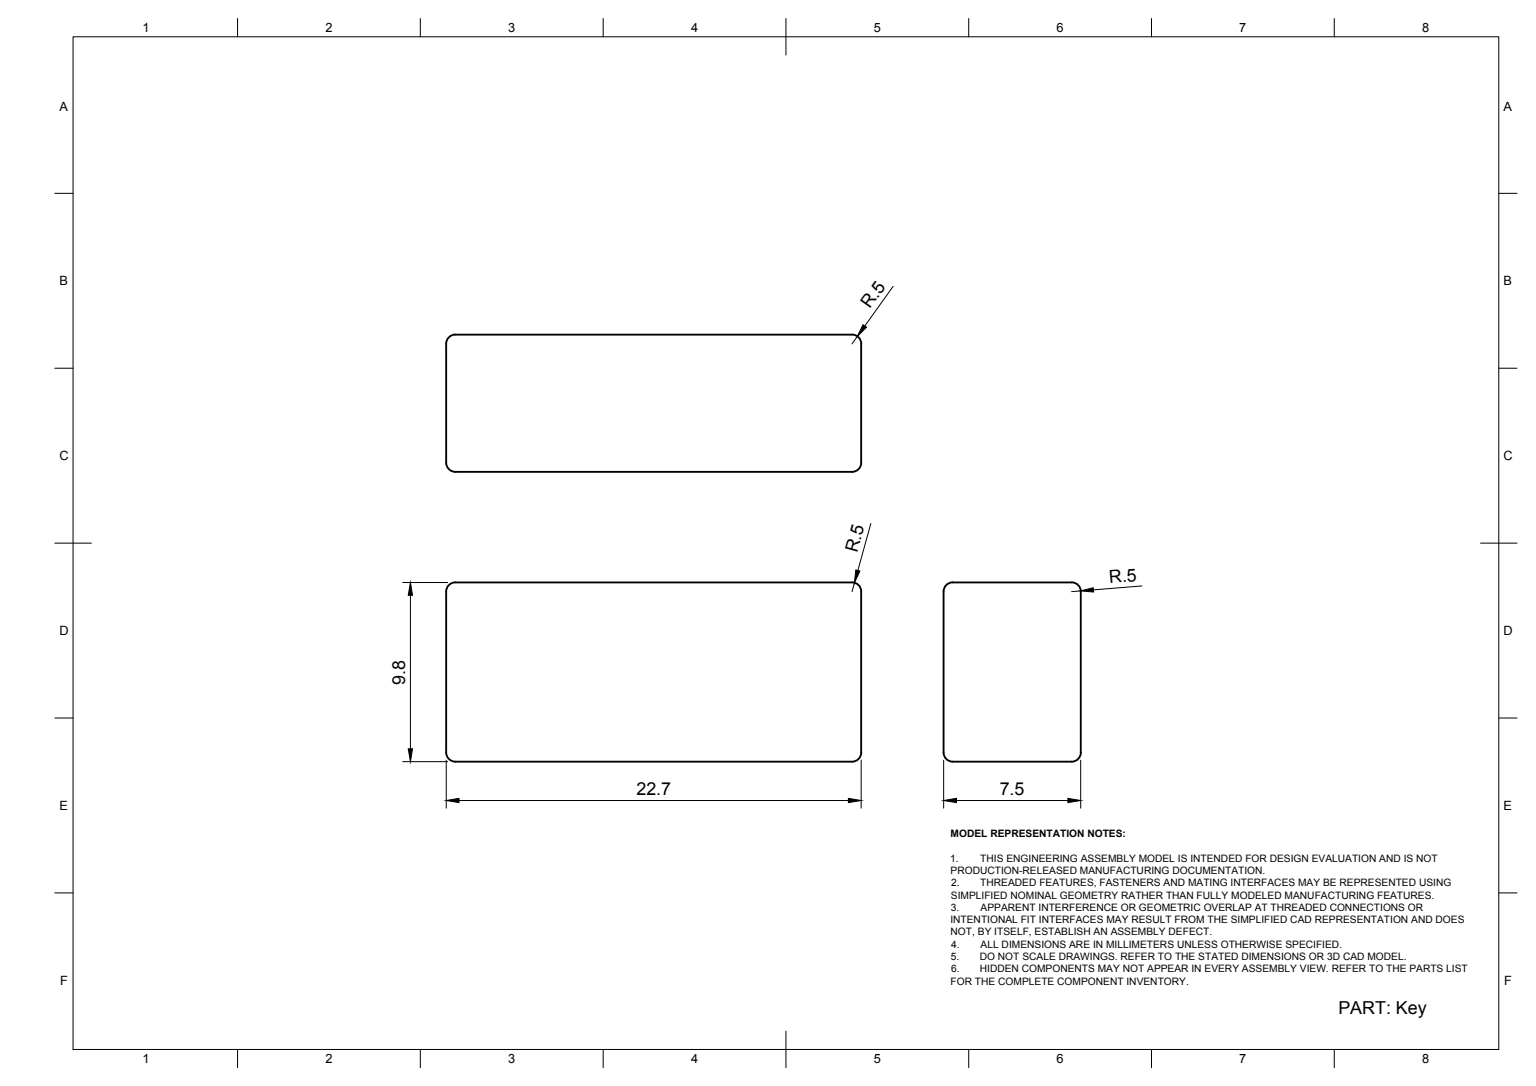
ISO-10303-21;
HEADER;
/* Generated by software containing ST-Developer
 * from STEP Tools, Inc. (www.steptools.com) 
 */

FILE_DESCRIPTION(
/* description */ ('STEP AP214'),
/* implementation_level */ '2;1');

FILE_NAME(
/* name */ 'Key.step',
/* time_stamp */ '2026-10-05T13:15:56-07:00',
/* author */ (''),
/* organization */ (''),
/* preprocessor_version */ 'ST-DEVELOPER v20.2',
/* originating_system */ 'Autodesk Translation Framework v15.15.0.0',
/* authorisation */ '');

FILE_SCHEMA (('AUTOMOTIVE_DESIGN { 1 0 10303 214 3 1 1 }'));
ENDSEC;

DATA;
#10=MECHANICAL_DESIGN_GEOMETRIC_PRESENTATION_REPRESENTATION('',(#1350),#37881);
#175=SPHERICAL_SURFACE('',#11699,0.5);
#176=SPHERICAL_SURFACE('',#11702,0.5);
#177=SPHERICAL_SURFACE('',#11719,0.5);
#178=SPHERICAL_SURFACE('',#11721,0.5);
#179=SPHERICAL_SURFACE('',#11723,0.5);
#180=SPHERICAL_SURFACE('',#11725,0.5);
#181=SPHERICAL_SURFACE('',#11735,0.5);
#182=SPHERICAL_SURFACE('',#11737,0.5);
#1326=SHAPE_REPRESENTATION_RELATIONSHIP('SRR','None',#37959,#1338);
#1338=ADVANCED_BREP_SHAPE_REPRESENTATION('',(#1362),#37874);
#1350=STYLED_ITEM('',(#38023),#1362);
#1362=MANIFOLD_SOLID_BREP('Body1',#10824);
#1525=PLANE('',#11690);
#1526=PLANE('',#11691);
#1527=PLANE('',#11692);
#1528=PLANE('',#11693);
#1529=PLANE('',#11694);
#1530=PLANE('',#11695);
#2091=FACE_OUTER_BOUND('',#2756,.T.);
#2092=FACE_OUTER_BOUND('',#2757,.T.);
#2093=FACE_OUTER_BOUND('',#2758,.T.);
#2094=FACE_OUTER_BOUND('',#2759,.T.);
#2095=FACE_OUTER_BOUND('',#2760,.T.);
#2096=FACE_OUTER_BOUND('',#2761,.T.);
#2097=FACE_OUTER_BOUND('',#2762,.T.);
#2098=FACE_OUTER_BOUND('',#2763,.T.);
#2099=FACE_OUTER_BOUND('',#2764,.T.);
#2100=FACE_OUTER_BOUND('',#2765,.T.);
#2101=FACE_OUTER_BOUND('',#2766,.T.);
#2102=FACE_OUTER_BOUND('',#2767,.T.);
#2103=FACE_OUTER_BOUND('',#2768,.T.);
#2104=FACE_OUTER_BOUND('',#2769,.T.);
#2105=FACE_OUTER_BOUND('',#2770,.T.);
#2106=FACE_OUTER_BOUND('',#2771,.T.);
#2107=FACE_OUTER_BOUND('',#2772,.T.);
#2108=FACE_OUTER_BOUND('',#2773,.T.);
#2109=FACE_OUTER_BOUND('',#2774,.T.);
#2110=FACE_OUTER_BOUND('',#2775,.T.);
#2111=FACE_OUTER_BOUND('',#2776,.T.);
#2112=FACE_OUTER_BOUND('',#2777,.T.);
#2113=FACE_OUTER_BOUND('',#2778,.T.);
#2114=FACE_OUTER_BOUND('',#2779,.T.);
#2115=FACE_OUTER_BOUND('',#2780,.T.);
#2116=FACE_OUTER_BOUND('',#2781,.T.);
#2756=EDGE_LOOP('',(#9677,#9678,#9679,#9680));
#2757=EDGE_LOOP('',(#9681,#9682,#9683,#9684));
#2758=EDGE_LOOP('',(#9685,#9686,#9687,#9688));
#2759=EDGE_LOOP('',(#9689,#9690,#9691,#9692));
#2760=EDGE_LOOP('',(#9693,#9694,#9695,#9696));
#2761=EDGE_LOOP('',(#9697,#9698,#9699,#9700));
#2762=EDGE_LOOP('',(#9701,#9702,#9703,#9704));
#2763=EDGE_LOOP('',(#9705,#9706,#9707));
#2764=EDGE_LOOP('',(#9708,#9709,#9710));
#2765=EDGE_LOOP('',(#9711,#9712,#9713,#9714));
#2766=EDGE_LOOP('',(#9715,#9716,#9717,#9718));
#2767=EDGE_LOOP('',(#9719,#9720,#9721,#9722));
#2768=EDGE_LOOP('',(#9723,#9724,#9725,#9726));
#2769=EDGE_LOOP('',(#9727,#9728,#9729,#9730));
#2770=EDGE_LOOP('',(#9731,#9732,#9733,#9734));
#2771=EDGE_LOOP('',(#9735,#9736,#9737));
#2772=EDGE_LOOP('',(#9738,#9739,#9740));
#2773=EDGE_LOOP('',(#9741,#9742,#9743));
#2774=EDGE_LOOP('',(#9744,#9745,#9746));
#2775=EDGE_LOOP('',(#9747,#9748,#9749,#9750));
#2776=EDGE_LOOP('',(#9751,#9752,#9753,#9754));
#2777=EDGE_LOOP('',(#9755,#9756,#9757,#9758));
#2778=EDGE_LOOP('',(#9759,#9760,#9761,#9762));
#2779=EDGE_LOOP('',(#9763,#9764,#9765));
#2780=EDGE_LOOP('',(#9766,#9767,#9768));
#2781=EDGE_LOOP('',(#9769,#9770,#9771,#9772));
#3066=LINE('',#37442,#3367);
#3067=LINE('',#37444,#3368);
#3068=LINE('',#37446,#3369);
#3069=LINE('',#37447,#3370);
#3070=LINE('',#37451,#3371);
#3071=LINE('',#37453,#3372);
#3072=LINE('',#37455,#3373);
#3073=LINE('',#37456,#3374);
#3074=LINE('',#37460,#3375);
#3075=LINE('',#37462,#3376);
#3076=LINE('',#37464,#3377);
#3077=LINE('',#37465,#3378);
#3078=LINE('',#37469,#3379);
#3079=LINE('',#37471,#3380);
#3080=LINE('',#37473,#3381);
#3081=LINE('',#37474,#3382);
#3082=LINE('',#37478,#3383);
#3083=LINE('',#37480,#3384);
#3084=LINE('',#37482,#3385);
#3085=LINE('',#37483,#3386);
#3086=LINE('',#37487,#3387);
#3087=LINE('',#37489,#3388);
#3088=LINE('',#37491,#3389);
#3089=LINE('',#37492,#3390);
#3367=VECTOR('',#13539,1000.);
#3368=VECTOR('',#13540,1000.);
#3369=VECTOR('',#13541,1000.);
#3370=VECTOR('',#13542,1000.);
#3371=VECTOR('',#13545,1000.);
#3372=VECTOR('',#13546,1000.);
#3373=VECTOR('',#13547,1000.);
#3374=VECTOR('',#13548,1000.);
#3375=VECTOR('',#13551,1000.);
#3376=VECTOR('',#13552,1000.);
#3377=VECTOR('',#13553,1000.);
#3378=VECTOR('',#13554,1000.);
#3379=VECTOR('',#13557,1000.);
#3380=VECTOR('',#13558,1000.);
#3381=VECTOR('',#13559,1000.);
#3382=VECTOR('',#13560,1000.);
#3383=VECTOR('',#13563,1000.);
#3384=VECTOR('',#13564,1000.);
#3385=VECTOR('',#13565,1000.);
#3386=VECTOR('',#13566,1000.);
#3387=VECTOR('',#13569,1000.);
#3388=VECTOR('',#13570,1000.);
#3389=VECTOR('',#13571,1000.);
#3390=VECTOR('',#13572,1000.);
#3928=CIRCLE('',#11697,0.5);
#3929=CIRCLE('',#11698,0.5);
#3930=CIRCLE('',#11700,0.5);
#3931=CIRCLE('',#11701,0.5);
#3932=CIRCLE('',#11703,0.5);
#3933=CIRCLE('',#11704,0.5);
#3934=CIRCLE('',#11706,0.5);
#3935=CIRCLE('',#11708,0.5);
#3936=CIRCLE('',#11710,0.5);
#3937=CIRCLE('',#11711,0.5);
#3938=CIRCLE('',#11713,0.5);
#3939=CIRCLE('',#11715,0.5);
#3940=CIRCLE('',#11717,0.5);
#3941=CIRCLE('',#11718,0.5);
#3942=CIRCLE('',#11720,0.5);
#3943=CIRCLE('',#11722,0.5);
#3944=CIRCLE('',#11724,0.5);
#3945=CIRCLE('',#11726,0.5);
#3946=CIRCLE('',#11728,0.5);
#3947=CIRCLE('',#11730,0.5);
#3948=CIRCLE('',#11732,0.5);
#3949=CIRCLE('',#11734,0.5);
#3950=CIRCLE('',#11736,0.5);
#3951=CIRCLE('',#11738,0.5);
#4964=VERTEX_POINT('',#37440);
#4965=VERTEX_POINT('',#37441);
#4966=VERTEX_POINT('',#37443);
#4967=VERTEX_POINT('',#37445);
#4968=VERTEX_POINT('',#37449);
#4969=VERTEX_POINT('',#37450);
#4970=VERTEX_POINT('',#37452);
#4971=VERTEX_POINT('',#37454);
#4972=VERTEX_POINT('',#37458);
#4973=VERTEX_POINT('',#37459);
#4974=VERTEX_POINT('',#37461);
#4975=VERTEX_POINT('',#37463);
#4976=VERTEX_POINT('',#37467);
#4977=VERTEX_POINT('',#37468);
#4978=VERTEX_POINT('',#37470);
#4979=VERTEX_POINT('',#37472);
#4980=VERTEX_POINT('',#37476);
#4981=VERTEX_POINT('',#37477);
#4982=VERTEX_POINT('',#37479);
#4983=VERTEX_POINT('',#37481);
#4984=VERTEX_POINT('',#37485);
#4985=VERTEX_POINT('',#37486);
#4986=VERTEX_POINT('',#37488);
#4987=VERTEX_POINT('',#37490);
#6549=EDGE_CURVE('',#4964,#4965,#3066,.T.);
#6550=EDGE_CURVE('',#4965,#4966,#3067,.T.);
#6551=EDGE_CURVE('',#4966,#4967,#3068,.T.);
#6552=EDGE_CURVE('',#4967,#4964,#3069,.T.);
#6553=EDGE_CURVE('',#4968,#4969,#3070,.T.);
#6554=EDGE_CURVE('',#4969,#4970,#3071,.T.);
#6555=EDGE_CURVE('',#4970,#4971,#3072,.T.);
#6556=EDGE_CURVE('',#4971,#4968,#3073,.T.);
#6557=EDGE_CURVE('',#4972,#4973,#3074,.T.);
#6558=EDGE_CURVE('',#4973,#4974,#3075,.T.);
#6559=EDGE_CURVE('',#4974,#4975,#3076,.T.);
#6560=EDGE_CURVE('',#4975,#4972,#3077,.T.);
#6561=EDGE_CURVE('',#4976,#4977,#3078,.T.);
#6562=EDGE_CURVE('',#4977,#4978,#3079,.T.);
#6563=EDGE_CURVE('',#4978,#4979,#3080,.T.);
#6564=EDGE_CURVE('',#4979,#4976,#3081,.T.);
#6565=EDGE_CURVE('',#4980,#4981,#3082,.T.);
#6566=EDGE_CURVE('',#4981,#4982,#3083,.T.);
#6567=EDGE_CURVE('',#4982,#4983,#3084,.T.);
#6568=EDGE_CURVE('',#4983,#4980,#3085,.T.);
#6569=EDGE_CURVE('',#4984,#4985,#3086,.T.);
#6570=EDGE_CURVE('',#4985,#4986,#3087,.T.);
#6571=EDGE_CURVE('',#4986,#4987,#3088,.T.);
#6572=EDGE_CURVE('',#4987,#4984,#3089,.T.);
#6573=EDGE_CURVE('',#4965,#4986,#3928,.T.);
#6574=EDGE_CURVE('',#4987,#4964,#3929,.T.);
#6575=EDGE_CURVE('',#4965,#4970,#3930,.T.);
#6576=EDGE_CURVE('',#4970,#4986,#3931,.T.);
#6577=EDGE_CURVE('',#4987,#4979,#3932,.T.);
#6578=EDGE_CURVE('',#4979,#4964,#3933,.T.);
#6579=EDGE_CURVE('',#4971,#4985,#3934,.T.);
#6580=EDGE_CURVE('',#4966,#4969,#3935,.T.);
#6581=EDGE_CURVE('',#4967,#4980,#3936,.T.);
#6582=EDGE_CURVE('',#4981,#4966,#3937,.T.);
#6583=EDGE_CURVE('',#4976,#4967,#3938,.T.);
#6584=EDGE_CURVE('',#4984,#4978,#3939,.T.);
#6585=EDGE_CURVE('',#4985,#4974,#3940,.T.);
#6586=EDGE_CURVE('',#4975,#4984,#3941,.T.);
#6587=EDGE_CURVE('',#4971,#4974,#3942,.T.);
#6588=EDGE_CURVE('',#4981,#4969,#3943,.T.);
#6589=EDGE_CURVE('',#4976,#4980,#3944,.T.);
#6590=EDGE_CURVE('',#4975,#4978,#3945,.T.);
#6591=EDGE_CURVE('',#4968,#4973,#3946,.T.);
#6592=EDGE_CURVE('',#4982,#4968,#3947,.T.);
#6593=EDGE_CURVE('',#4977,#4983,#3948,.T.);
#6594=EDGE_CURVE('',#4972,#4977,#3949,.T.);
#6595=EDGE_CURVE('',#4982,#4973,#3950,.T.);
#6596=EDGE_CURVE('',#4972,#4983,#3951,.T.);
#9677=ORIENTED_EDGE('',*,*,#6549,.T.);
#9678=ORIENTED_EDGE('',*,*,#6550,.T.);
#9679=ORIENTED_EDGE('',*,*,#6551,.T.);
#9680=ORIENTED_EDGE('',*,*,#6552,.T.);
#9681=ORIENTED_EDGE('',*,*,#6553,.T.);
#9682=ORIENTED_EDGE('',*,*,#6554,.T.);
#9683=ORIENTED_EDGE('',*,*,#6555,.T.);
#9684=ORIENTED_EDGE('',*,*,#6556,.T.);
#9685=ORIENTED_EDGE('',*,*,#6557,.T.);
#9686=ORIENTED_EDGE('',*,*,#6558,.T.);
#9687=ORIENTED_EDGE('',*,*,#6559,.T.);
#9688=ORIENTED_EDGE('',*,*,#6560,.T.);
#9689=ORIENTED_EDGE('',*,*,#6561,.T.);
#9690=ORIENTED_EDGE('',*,*,#6562,.T.);
#9691=ORIENTED_EDGE('',*,*,#6563,.T.);
#9692=ORIENTED_EDGE('',*,*,#6564,.T.);
#9693=ORIENTED_EDGE('',*,*,#6565,.T.);
#9694=ORIENTED_EDGE('',*,*,#6566,.T.);
#9695=ORIENTED_EDGE('',*,*,#6567,.T.);
#9696=ORIENTED_EDGE('',*,*,#6568,.T.);
#9697=ORIENTED_EDGE('',*,*,#6569,.T.);
#9698=ORIENTED_EDGE('',*,*,#6570,.T.);
#9699=ORIENTED_EDGE('',*,*,#6571,.T.);
#9700=ORIENTED_EDGE('',*,*,#6572,.T.);
#9701=ORIENTED_EDGE('',*,*,#6573,.F.);
#9702=ORIENTED_EDGE('',*,*,#6549,.F.);
#9703=ORIENTED_EDGE('',*,*,#6574,.F.);
#9704=ORIENTED_EDGE('',*,*,#6571,.F.);
#9705=ORIENTED_EDGE('',*,*,#6575,.F.);
#9706=ORIENTED_EDGE('',*,*,#6573,.T.);
#9707=ORIENTED_EDGE('',*,*,#6576,.F.);
#9708=ORIENTED_EDGE('',*,*,#6577,.F.);
#9709=ORIENTED_EDGE('',*,*,#6574,.T.);
#9710=ORIENTED_EDGE('',*,*,#6578,.F.);
#9711=ORIENTED_EDGE('',*,*,#6576,.T.);
#9712=ORIENTED_EDGE('',*,*,#6570,.F.);
#9713=ORIENTED_EDGE('',*,*,#6579,.F.);
#9714=ORIENTED_EDGE('',*,*,#6555,.F.);
#9715=ORIENTED_EDGE('',*,*,#6575,.T.);
#9716=ORIENTED_EDGE('',*,*,#6554,.F.);
#9717=ORIENTED_EDGE('',*,*,#6580,.F.);
#9718=ORIENTED_EDGE('',*,*,#6550,.F.);
#9719=ORIENTED_EDGE('',*,*,#6581,.F.);
#9720=ORIENTED_EDGE('',*,*,#6551,.F.);
#9721=ORIENTED_EDGE('',*,*,#6582,.F.);
#9722=ORIENTED_EDGE('',*,*,#6565,.F.);
#9723=ORIENTED_EDGE('',*,*,#6578,.T.);
#9724=ORIENTED_EDGE('',*,*,#6552,.F.);
#9725=ORIENTED_EDGE('',*,*,#6583,.F.);
#9726=ORIENTED_EDGE('',*,*,#6564,.F.);
#9727=ORIENTED_EDGE('',*,*,#6577,.T.);
#9728=ORIENTED_EDGE('',*,*,#6563,.F.);
#9729=ORIENTED_EDGE('',*,*,#6584,.F.);
#9730=ORIENTED_EDGE('',*,*,#6572,.F.);
#9731=ORIENTED_EDGE('',*,*,#6585,.F.);
#9732=ORIENTED_EDGE('',*,*,#6569,.F.);
#9733=ORIENTED_EDGE('',*,*,#6586,.F.);
#9734=ORIENTED_EDGE('',*,*,#6559,.F.);
#9735=ORIENTED_EDGE('',*,*,#6579,.T.);
#9736=ORIENTED_EDGE('',*,*,#6585,.T.);
#9737=ORIENTED_EDGE('',*,*,#6587,.F.);
#9738=ORIENTED_EDGE('',*,*,#6582,.T.);
#9739=ORIENTED_EDGE('',*,*,#6580,.T.);
#9740=ORIENTED_EDGE('',*,*,#6588,.F.);
#9741=ORIENTED_EDGE('',*,*,#6583,.T.);
#9742=ORIENTED_EDGE('',*,*,#6581,.T.);
#9743=ORIENTED_EDGE('',*,*,#6589,.F.);
#9744=ORIENTED_EDGE('',*,*,#6586,.T.);
#9745=ORIENTED_EDGE('',*,*,#6584,.T.);
#9746=ORIENTED_EDGE('',*,*,#6590,.F.);
#9747=ORIENTED_EDGE('',*,*,#6587,.T.);
#9748=ORIENTED_EDGE('',*,*,#6558,.F.);
#9749=ORIENTED_EDGE('',*,*,#6591,.F.);
#9750=ORIENTED_EDGE('',*,*,#6556,.F.);
#9751=ORIENTED_EDGE('',*,*,#6588,.T.);
#9752=ORIENTED_EDGE('',*,*,#6553,.F.);
#9753=ORIENTED_EDGE('',*,*,#6592,.F.);
#9754=ORIENTED_EDGE('',*,*,#6566,.F.);
#9755=ORIENTED_EDGE('',*,*,#6589,.T.);
#9756=ORIENTED_EDGE('',*,*,#6568,.F.);
#9757=ORIENTED_EDGE('',*,*,#6593,.F.);
#9758=ORIENTED_EDGE('',*,*,#6561,.F.);
#9759=ORIENTED_EDGE('',*,*,#6590,.T.);
#9760=ORIENTED_EDGE('',*,*,#6562,.F.);
#9761=ORIENTED_EDGE('',*,*,#6594,.F.);
#9762=ORIENTED_EDGE('',*,*,#6560,.F.);
#9763=ORIENTED_EDGE('',*,*,#6592,.T.);
#9764=ORIENTED_EDGE('',*,*,#6591,.T.);
#9765=ORIENTED_EDGE('',*,*,#6595,.F.);
#9766=ORIENTED_EDGE('',*,*,#6594,.T.);
#9767=ORIENTED_EDGE('',*,*,#6593,.T.);
#9768=ORIENTED_EDGE('',*,*,#6596,.F.);
#9769=ORIENTED_EDGE('',*,*,#6595,.T.);
#9770=ORIENTED_EDGE('',*,*,#6557,.F.);
#9771=ORIENTED_EDGE('',*,*,#6596,.T.);
#9772=ORIENTED_EDGE('',*,*,#6567,.F.);
#10177=CYLINDRICAL_SURFACE('',#11696,0.5);
#10178=CYLINDRICAL_SURFACE('',#11705,0.5);
#10179=CYLINDRICAL_SURFACE('',#11707,0.5);
#10180=CYLINDRICAL_SURFACE('',#11709,0.5);
#10181=CYLINDRICAL_SURFACE('',#11712,0.5);
#10182=CYLINDRICAL_SURFACE('',#11714,0.5);
#10183=CYLINDRICAL_SURFACE('',#11716,0.5);
#10184=CYLINDRICAL_SURFACE('',#11727,0.5);
#10185=CYLINDRICAL_SURFACE('',#11729,0.5);
#10186=CYLINDRICAL_SURFACE('',#11731,0.5);
#10187=CYLINDRICAL_SURFACE('',#11733,0.5);
#10188=CYLINDRICAL_SURFACE('',#11739,0.5);
#10736=ADVANCED_FACE('',(#2091),#1525,.F.);
#10737=ADVANCED_FACE('',(#2092),#1526,.F.);
#10738=ADVANCED_FACE('',(#2093),#1527,.F.);
#10739=ADVANCED_FACE('',(#2094),#1528,.F.);
#10740=ADVANCED_FACE('',(#2095),#1529,.F.);
#10741=ADVANCED_FACE('',(#2096),#1530,.T.);
#10742=ADVANCED_FACE('',(#2097),#10177,.T.);
#10743=ADVANCED_FACE('',(#2098),#175,.T.);
#10744=ADVANCED_FACE('',(#2099),#176,.T.);
#10745=ADVANCED_FACE('',(#2100),#10178,.T.);
#10746=ADVANCED_FACE('',(#2101),#10179,.T.);
#10747=ADVANCED_FACE('',(#2102),#10180,.T.);
#10748=ADVANCED_FACE('',(#2103),#10181,.T.);
#10749=ADVANCED_FACE('',(#2104),#10182,.T.);
#10750=ADVANCED_FACE('',(#2105),#10183,.T.);
#10751=ADVANCED_FACE('',(#2106),#177,.T.);
#10752=ADVANCED_FACE('',(#2107),#178,.T.);
#10753=ADVANCED_FACE('',(#2108),#179,.T.);
#10754=ADVANCED_FACE('',(#2109),#180,.T.);
#10755=ADVANCED_FACE('',(#2110),#10184,.T.);
#10756=ADVANCED_FACE('',(#2111),#10185,.T.);
#10757=ADVANCED_FACE('',(#2112),#10186,.T.);
#10758=ADVANCED_FACE('',(#2113),#10187,.T.);
#10759=ADVANCED_FACE('',(#2114),#181,.T.);
#10760=ADVANCED_FACE('',(#2115),#182,.T.);
#10761=ADVANCED_FACE('',(#2116),#10188,.T.);
#10824=CLOSED_SHELL('',(#10736,#10737,#10738,#10739,#10740,#10741,#10742,
#10743,#10744,#10745,#10746,#10747,#10748,#10749,#10750,#10751,#10752,#10753,
#10754,#10755,#10756,#10757,#10758,#10759,#10760,#10761));
#11689=AXIS2_PLACEMENT_3D('',#37438,#13535,#13536);
#11690=AXIS2_PLACEMENT_3D('',#37439,#13537,#13538);
#11691=AXIS2_PLACEMENT_3D('',#37448,#13543,#13544);
#11692=AXIS2_PLACEMENT_3D('',#37457,#13549,#13550);
#11693=AXIS2_PLACEMENT_3D('',#37466,#13555,#13556);
#11694=AXIS2_PLACEMENT_3D('',#37475,#13561,#13562);
#11695=AXIS2_PLACEMENT_3D('',#37484,#13567,#13568);
#11696=AXIS2_PLACEMENT_3D('',#37493,#13573,#13574);
#11697=AXIS2_PLACEMENT_3D('',#37494,#13575,#13576);
#11698=AXIS2_PLACEMENT_3D('',#37495,#13577,#13578);
#11699=AXIS2_PLACEMENT_3D('',#37496,#13579,#13580);
#11700=AXIS2_PLACEMENT_3D('',#37497,#13581,#13582);
#11701=AXIS2_PLACEMENT_3D('',#37498,#13583,#13584);
#11702=AXIS2_PLACEMENT_3D('',#37499,#13585,#13586);
#11703=AXIS2_PLACEMENT_3D('',#37500,#13587,#13588);
#11704=AXIS2_PLACEMENT_3D('',#37501,#13589,#13590);
#11705=AXIS2_PLACEMENT_3D('',#37502,#13591,#13592);
#11706=AXIS2_PLACEMENT_3D('',#37503,#13593,#13594);
#11707=AXIS2_PLACEMENT_3D('',#37504,#13595,#13596);
#11708=AXIS2_PLACEMENT_3D('',#37505,#13597,#13598);
#11709=AXIS2_PLACEMENT_3D('',#37506,#13599,#13600);
#11710=AXIS2_PLACEMENT_3D('',#37507,#13601,#13602);
#11711=AXIS2_PLACEMENT_3D('',#37508,#13603,#13604);
#11712=AXIS2_PLACEMENT_3D('',#37509,#13605,#13606);
#11713=AXIS2_PLACEMENT_3D('',#37510,#13607,#13608);
#11714=AXIS2_PLACEMENT_3D('',#37511,#13609,#13610);
#11715=AXIS2_PLACEMENT_3D('',#37512,#13611,#13612);
#11716=AXIS2_PLACEMENT_3D('',#37513,#13613,#13614);
#11717=AXIS2_PLACEMENT_3D('',#37514,#13615,#13616);
#11718=AXIS2_PLACEMENT_3D('',#37515,#13617,#13618);
#11719=AXIS2_PLACEMENT_3D('',#37516,#13619,#13620);
#11720=AXIS2_PLACEMENT_3D('',#37517,#13621,#13622);
#11721=AXIS2_PLACEMENT_3D('',#37518,#13623,#13624);
#11722=AXIS2_PLACEMENT_3D('',#37519,#13625,#13626);
#11723=AXIS2_PLACEMENT_3D('',#37520,#13627,#13628);
#11724=AXIS2_PLACEMENT_3D('',#37521,#13629,#13630);
#11725=AXIS2_PLACEMENT_3D('',#37522,#13631,#13632);
#11726=AXIS2_PLACEMENT_3D('',#37523,#13633,#13634);
#11727=AXIS2_PLACEMENT_3D('',#37524,#13635,#13636);
#11728=AXIS2_PLACEMENT_3D('',#37525,#13637,#13638);
#11729=AXIS2_PLACEMENT_3D('',#37526,#13639,#13640);
#11730=AXIS2_PLACEMENT_3D('',#37527,#13641,#13642);
#11731=AXIS2_PLACEMENT_3D('',#37528,#13643,#13644);
#11732=AXIS2_PLACEMENT_3D('',#37529,#13645,#13646);
#11733=AXIS2_PLACEMENT_3D('',#37530,#13647,#13648);
#11734=AXIS2_PLACEMENT_3D('',#37531,#13649,#13650);
#11735=AXIS2_PLACEMENT_3D('',#37532,#13651,#13652);
#11736=AXIS2_PLACEMENT_3D('',#37533,#13653,#13654);
#11737=AXIS2_PLACEMENT_3D('',#37534,#13655,#13656);
#11738=AXIS2_PLACEMENT_3D('',#37535,#13657,#13658);
#11739=AXIS2_PLACEMENT_3D('',#37536,#13659,#13660);
#13535=DIRECTION('axis',(0.,0.,1.));
#13536=DIRECTION('refdir',(1.,0.,0.));
#13537=DIRECTION('center_axis',(-1.,0.,0.));
#13538=DIRECTION('ref_axis',(0.,0.,1.));
#13539=DIRECTION('',(0.,1.,0.));
#13540=DIRECTION('',(0.,0.,1.));
#13541=DIRECTION('',(0.,-1.,0.));
#13542=DIRECTION('',(0.,0.,-1.));
#13543=DIRECTION('center_axis',(0.,-1.,0.));
#13544=DIRECTION('ref_axis',(0.,0.,-1.));
#13545=DIRECTION('',(1.,0.,0.));
#13546=DIRECTION('',(0.,0.,-1.));
#13547=DIRECTION('',(-1.,0.,0.));
#13548=DIRECTION('',(0.,0.,1.));
#13549=DIRECTION('center_axis',(1.,0.,0.));
#13550=DIRECTION('ref_axis',(0.,0.,-1.));
#13551=DIRECTION('',(0.,1.,0.));
#13552=DIRECTION('',(0.,0.,-1.));
#13553=DIRECTION('',(0.,-1.,0.));
#13554=DIRECTION('',(0.,0.,1.));
#13555=DIRECTION('center_axis',(-4.42531498973675E-17,1.,0.));
#13556=DIRECTION('ref_axis',(-1.,-4.42531498973675E-17,0.));
#13557=DIRECTION('',(-1.,-4.42531498973675E-17,0.));
#13558=DIRECTION('',(0.,0.,-1.));
#13559=DIRECTION('',(1.,4.42531498973675E-17,0.));
#13560=DIRECTION('',(0.,0.,1.));
#13561=DIRECTION('center_axis',(0.,0.,-1.));
#13562=DIRECTION('ref_axis',(-1.,0.,0.));
#13563=DIRECTION('',(0.,1.,0.));
#13564=DIRECTION('',(-1.,0.,0.));
#13565=DIRECTION('',(0.,-1.,0.));
#13566=DIRECTION('',(1.,4.42531498973675E-17,0.));
#13567=DIRECTION('center_axis',(0.,0.,-1.));
#13568=DIRECTION('ref_axis',(-1.,0.,0.));
#13569=DIRECTION('',(0.,1.,0.));
#13570=DIRECTION('',(1.,0.,0.));
#13571=DIRECTION('',(0.,-1.,0.));
#13572=DIRECTION('',(-1.,-4.42531498973675E-17,0.));
#13573=DIRECTION('center_axis',(0.,-1.,0.));
#13574=DIRECTION('ref_axis',(0.,0.,-1.));
#13575=DIRECTION('center_axis',(0.,1.,0.));
#13576=DIRECTION('ref_axis',(0.,0.,1.));
#13577=DIRECTION('center_axis',(0.,-1.,0.));
#13578=DIRECTION('ref_axis',(0.,0.,-1.));
#13579=DIRECTION('center_axis',(0.,1.,0.));
#13580=DIRECTION('ref_axis',(-1.,0.,0.));
#13581=DIRECTION('center_axis',(0.,0.,1.));
#13582=DIRECTION('ref_axis',(-1.,0.,0.));
#13583=DIRECTION('center_axis',(-1.,1.73472347597681E-15,0.));
#13584=DIRECTION('ref_axis',(1.73472347597681E-15,1.,0.));
#13585=DIRECTION('center_axis',(0.,1.,-1.11022302462516E-16));
#13586=DIRECTION('ref_axis',(1.77635683940025E-15,0.,-1.));
#13587=DIRECTION('center_axis',(-1.,0.,0.));
#13588=DIRECTION('ref_axis',(0.,0.,-1.));
#13589=DIRECTION('center_axis',(0.,0.,1.));
#13590=DIRECTION('ref_axis',(-1.,0.,0.));
#13591=DIRECTION('center_axis',(1.,0.,0.));
#13592=DIRECTION('ref_axis',(0.,0.,-1.));
#13593=DIRECTION('center_axis',(-1.,0.,0.));
#13594=DIRECTION('ref_axis',(0.,0.,1.));
#13595=DIRECTION('center_axis',(0.,0.,-1.));
#13596=DIRECTION('ref_axis',(-1.,0.,0.));
#13597=DIRECTION('center_axis',(0.,0.,1.));
#13598=DIRECTION('ref_axis',(1.,0.,0.));
#13599=DIRECTION('center_axis',(0.,1.,0.));
#13600=DIRECTION('ref_axis',(0.,0.,1.));
#13601=DIRECTION('center_axis',(0.,-1.,0.));
#13602=DIRECTION('ref_axis',(0.,0.,-1.));
#13603=DIRECTION('center_axis',(0.,1.,0.));
#13604=DIRECTION('ref_axis',(0.,0.,1.));
#13605=DIRECTION('center_axis',(0.,0.,-1.));
#13606=DIRECTION('ref_axis',(-1.,0.,0.));
#13607=DIRECTION('center_axis',(0.,0.,1.));
#13608=DIRECTION('ref_axis',(1.,0.,0.));
#13609=DIRECTION('center_axis',(-1.,-4.42531498973675E-17,0.));
#13610=DIRECTION('ref_axis',(4.42531498973675E-17,-1.,0.));
#13611=DIRECTION('center_axis',(-1.,0.,0.));
#13612=DIRECTION('ref_axis',(0.,0.,1.));
#13613=DIRECTION('center_axis',(0.,1.,0.));
#13614=DIRECTION('ref_axis',(0.,0.,1.));
#13615=DIRECTION('center_axis',(-8.67361737988404E-16,1.,0.));
#13616=DIRECTION('ref_axis',(-1.,-8.67361737988404E-16,0.));
#13617=DIRECTION('center_axis',(0.,-1.,0.));
#13618=DIRECTION('ref_axis',(0.,0.,-1.));
#13619=DIRECTION('center_axis',(0.,1.,0.));
#13620=DIRECTION('ref_axis',(-1.,0.,0.));
#13621=DIRECTION('center_axis',(0.,0.,1.));
#13622=DIRECTION('ref_axis',(-1.,0.,0.));
#13623=DIRECTION('center_axis',(0.,1.,0.));
#13624=DIRECTION('ref_axis',(0.,0.,-1.));
#13625=DIRECTION('center_axis',(-1.,0.,-1.73472347597681E-15));
#13626=DIRECTION('ref_axis',(1.73472347597681E-15,0.,-1.));
#13627=DIRECTION('center_axis',(0.,1.,0.));
#13628=DIRECTION('ref_axis',(0.,0.,-1.));
#13629=DIRECTION('center_axis',(-1.,0.,0.));
#13630=DIRECTION('ref_axis',(0.,0.,-1.));
#13631=DIRECTION('center_axis',(0.,1.,0.));
#13632=DIRECTION('ref_axis',(-1.,0.,0.));
#13633=DIRECTION('center_axis',(0.,0.,1.));
#13634=DIRECTION('ref_axis',(-1.,0.,0.));
#13635=DIRECTION('center_axis',(0.,0.,-1.));
#13636=DIRECTION('ref_axis',(-1.,0.,0.));
#13637=DIRECTION('center_axis',(0.,0.,1.));
#13638=DIRECTION('ref_axis',(1.,0.,0.));
#13639=DIRECTION('center_axis',(-1.,0.,0.));
#13640=DIRECTION('ref_axis',(0.,0.,1.));
#13641=DIRECTION('center_axis',(-1.,0.,0.));
#13642=DIRECTION('ref_axis',(0.,0.,1.));
#13643=DIRECTION('center_axis',(1.,4.42531498973675E-17,0.));
#13644=DIRECTION('ref_axis',(-4.42531498973675E-17,1.,0.));
#13645=DIRECTION('center_axis',(-1.,0.,0.));
#13646=DIRECTION('ref_axis',(0.,0.,1.));
#13647=DIRECTION('center_axis',(0.,0.,-1.));
#13648=DIRECTION('ref_axis',(-1.,0.,0.));
#13649=DIRECTION('center_axis',(0.,0.,1.));
#13650=DIRECTION('ref_axis',(1.,0.,0.));
#13651=DIRECTION('center_axis',(1.,0.,0.));
#13652=DIRECTION('ref_axis',(0.,0.,1.));
#13653=DIRECTION('center_axis',(0.,-1.,8.67361737988403E-16));
#13654=DIRECTION('ref_axis',(0.,8.67361737988403E-16,1.));
#13655=DIRECTION('center_axis',(1.,0.,0.));
#13656=DIRECTION('ref_axis',(0.,0.,-1.));
#13657=DIRECTION('center_axis',(0.,1.,0.));
#13658=DIRECTION('ref_axis',(0.,0.,-1.));
#13659=DIRECTION('center_axis',(0.,-1.,0.));
#13660=DIRECTION('ref_axis',(0.,0.,-1.));
#37438=CARTESIAN_POINT('',(0.,0.,0.));
#37439=CARTESIAN_POINT('Origin',(4.9,-3.75,22.7));
#37440=CARTESIAN_POINT('',(4.9,-3.25,0.5));
#37441=CARTESIAN_POINT('',(4.9,3.25,0.5));
#37442=CARTESIAN_POINT('',(4.9,3.75,0.5));
#37443=CARTESIAN_POINT('',(4.9,3.25,22.2));
#37444=CARTESIAN_POINT('',(4.9,3.25,22.7));
#37445=CARTESIAN_POINT('',(4.9,-3.25,22.2));
#37446=CARTESIAN_POINT('',(4.9,-3.75,22.2));
#37447=CARTESIAN_POINT('',(4.9,-3.25,22.7));
#37448=CARTESIAN_POINT('Origin',(-4.9,3.75,22.7));
#37449=CARTESIAN_POINT('',(-4.4,3.75,22.2));
#37450=CARTESIAN_POINT('',(4.4,3.75,22.2));
#37451=CARTESIAN_POINT('',(-4.9,3.75,22.2));
#37452=CARTESIAN_POINT('',(4.4,3.75,0.5));
#37453=CARTESIAN_POINT('',(4.4,3.75,22.7));
#37454=CARTESIAN_POINT('',(-4.4,3.75,0.5));
#37455=CARTESIAN_POINT('',(-4.9,3.75,0.5));
#37456=CARTESIAN_POINT('',(-4.4,3.75,22.7));
#37457=CARTESIAN_POINT('Origin',(-4.9,-3.75,22.7));
#37458=CARTESIAN_POINT('',(-4.9,-3.25,22.2));
#37459=CARTESIAN_POINT('',(-4.9,3.25,22.2));
#37460=CARTESIAN_POINT('',(-4.9,-3.75,22.2));
#37461=CARTESIAN_POINT('',(-4.9,3.25,0.5));
#37462=CARTESIAN_POINT('',(-4.9,3.25,22.7));
#37463=CARTESIAN_POINT('',(-4.9,-3.25,0.5));
#37464=CARTESIAN_POINT('',(-4.9,-3.75,0.5));
#37465=CARTESIAN_POINT('',(-4.9,-3.25,22.7));
#37466=CARTESIAN_POINT('Origin',(-4.9,-3.75,22.7));
#37467=CARTESIAN_POINT('',(4.4,-3.75,22.2));
#37468=CARTESIAN_POINT('',(-4.4,-3.75,22.2));
#37469=CARTESIAN_POINT('',(-4.9,-3.75,22.2));
#37470=CARTESIAN_POINT('',(-4.4,-3.75,0.5));
#37471=CARTESIAN_POINT('',(-4.4,-3.75,22.7));
#37472=CARTESIAN_POINT('',(4.4,-3.75,0.5));
#37473=CARTESIAN_POINT('',(4.9,-3.75,0.5));
#37474=CARTESIAN_POINT('',(4.4,-3.75,22.7));
#37475=CARTESIAN_POINT('Origin',(0.,0.,22.7));
#37476=CARTESIAN_POINT('',(4.4,-3.25,22.7));
#37477=CARTESIAN_POINT('',(4.4,3.25,22.7));
#37478=CARTESIAN_POINT('',(4.4,0.,22.7));
#37479=CARTESIAN_POINT('',(-4.4,3.25,22.7));
#37480=CARTESIAN_POINT('',(0.,3.25,22.7));
#37481=CARTESIAN_POINT('',(-4.4,-3.25,22.7));
#37482=CARTESIAN_POINT('',(-4.4,0.,22.7));
#37483=CARTESIAN_POINT('',(1.43822737166444E-16,-3.25,22.7));
#37484=CARTESIAN_POINT('Origin',(0.,0.,0.));
#37485=CARTESIAN_POINT('',(-4.4,-3.25,0.));
#37486=CARTESIAN_POINT('',(-4.4,3.25,0.));
#37487=CARTESIAN_POINT('',(-4.4,3.75,0.));
#37488=CARTESIAN_POINT('',(4.4,3.25,0.));
#37489=CARTESIAN_POINT('',(4.9,3.25,0.));
#37490=CARTESIAN_POINT('',(4.4,-3.25,0.));
#37491=CARTESIAN_POINT('',(4.4,-3.75,0.));
#37492=CARTESIAN_POINT('',(-4.9,-3.25,0.));
#37493=CARTESIAN_POINT('Origin',(4.4,-3.75,0.5));
#37494=CARTESIAN_POINT('Origin',(4.4,3.25,0.5));
#37495=CARTESIAN_POINT('Origin',(4.4,-3.25,0.5));
#37496=CARTESIAN_POINT('Origin',(4.4,3.25,0.5));
#37497=CARTESIAN_POINT('Origin',(4.4,3.25,0.5));
#37498=CARTESIAN_POINT('Origin',(4.4,3.25,0.5));
#37499=CARTESIAN_POINT('Origin',(4.4,-3.25,0.5));
#37500=CARTESIAN_POINT('Origin',(4.4,-3.25,0.5));
#37501=CARTESIAN_POINT('Origin',(4.4,-3.25,0.5));
#37502=CARTESIAN_POINT('Origin',(-4.9,3.25,0.5));
#37503=CARTESIAN_POINT('Origin',(-4.4,3.25,0.5));
#37504=CARTESIAN_POINT('Origin',(4.4,3.25,22.7));
#37505=CARTESIAN_POINT('Origin',(4.4,3.25,22.2));
#37506=CARTESIAN_POINT('Origin',(4.4,0.,22.2));
#37507=CARTESIAN_POINT('Origin',(4.4,-3.25,22.2));
#37508=CARTESIAN_POINT('Origin',(4.4,3.25,22.2));
#37509=CARTESIAN_POINT('Origin',(4.4,-3.25,22.7));
#37510=CARTESIAN_POINT('Origin',(4.4,-3.25,22.2));
#37511=CARTESIAN_POINT('Origin',(-4.9,-3.25,0.5));
#37512=CARTESIAN_POINT('Origin',(-4.4,-3.25,0.5));
#37513=CARTESIAN_POINT('Origin',(-4.4,-3.75,0.5));
#37514=CARTESIAN_POINT('Origin',(-4.4,3.25,0.5));
#37515=CARTESIAN_POINT('Origin',(-4.4,-3.25,0.5));
#37516=CARTESIAN_POINT('Origin',(-4.4,3.25,0.5));
#37517=CARTESIAN_POINT('Origin',(-4.4,3.25,0.5));
#37518=CARTESIAN_POINT('Origin',(4.4,3.25,22.2));
#37519=CARTESIAN_POINT('Origin',(4.4,3.25,22.2));
#37520=CARTESIAN_POINT('Origin',(4.4,-3.25,22.2));
#37521=CARTESIAN_POINT('Origin',(4.4,-3.25,22.2));
#37522=CARTESIAN_POINT('Origin',(-4.4,-3.25,0.5));
#37523=CARTESIAN_POINT('Origin',(-4.4,-3.25,0.5));
#37524=CARTESIAN_POINT('Origin',(-4.4,3.25,22.7));
#37525=CARTESIAN_POINT('Origin',(-4.4,3.25,22.2));
#37526=CARTESIAN_POINT('Origin',(0.,3.25,22.2));
#37527=CARTESIAN_POINT('Origin',(-4.4,3.25,22.2));
#37528=CARTESIAN_POINT('Origin',(1.43822737166444E-16,-3.25,22.2));
#37529=CARTESIAN_POINT('Origin',(-4.4,-3.25,22.2));
#37530=CARTESIAN_POINT('Origin',(-4.4,-3.25,22.7));
#37531=CARTESIAN_POINT('Origin',(-4.4,-3.25,22.2));
#37532=CARTESIAN_POINT('Origin',(-4.4,3.25,22.2));
#37533=CARTESIAN_POINT('Origin',(-4.4,3.25,22.2));
#37534=CARTESIAN_POINT('Origin',(-4.4,-3.25,22.2));
#37535=CARTESIAN_POINT('Origin',(-4.4,-3.25,22.2));
#37536=CARTESIAN_POINT('Origin',(-4.4,0.,22.2));
#37860=UNCERTAINTY_MEASURE_WITH_UNIT(LENGTH_MEASURE(0.01),#37882,
'DISTANCE_ACCURACY_VALUE',
'Maximum model space distance between geometric entities at asserted c
onnectivities');
#37867=UNCERTAINTY_MEASURE_WITH_UNIT(LENGTH_MEASURE(0.01),#37882,
'DISTANCE_ACCURACY_VALUE',
'Maximum model space distance between geometric entities at asserted c
onnectivities');
#37874=(
GEOMETRIC_REPRESENTATION_CONTEXT(3)
GLOBAL_UNCERTAINTY_ASSIGNED_CONTEXT((#37860))
GLOBAL_UNIT_ASSIGNED_CONTEXT((#37882,#37884,#37885))
REPRESENTATION_CONTEXT('','3D')
);
#37881=(
GEOMETRIC_REPRESENTATION_CONTEXT(3)
GLOBAL_UNCERTAINTY_ASSIGNED_CONTEXT((#37867))
GLOBAL_UNIT_ASSIGNED_CONTEXT((#37882,#37884,#37885))
REPRESENTATION_CONTEXT('','3D')
);
#37882=(
LENGTH_UNIT()
NAMED_UNIT(*)
SI_UNIT(.MILLI.,.METRE.)
);
#37884=(
NAMED_UNIT(*)
PLANE_ANGLE_UNIT()
SI_UNIT($,.RADIAN.)
);
#37885=(
NAMED_UNIT(*)
SI_UNIT($,.STERADIAN.)
SOLID_ANGLE_UNIT()
);
#37892=SHAPE_DEFINITION_REPRESENTATION(#37905,#37959);
#37905=PRODUCT_DEFINITION_SHAPE('',$,#37973);
#37959=SHAPE_REPRESENTATION('',(#11689),#37874);
#37966=PRODUCT_DEFINITION_CONTEXT('part definition',#38007,'design');
#37973=PRODUCT_DEFINITION('PS08','Key',#37986,#37966);
#37986=PRODUCT_DEFINITION_FORMATION('',$,#38015);
#38007=APPLICATION_CONTEXT(
'Core Data for Automotive Mechanical Design Process');
#38008=PRODUCT_CONTEXT('part definition',#38007,'mechanical');
#38015=PRODUCT('PS08','Key',$,(#38008));
#38023=PRESENTATION_STYLE_ASSIGNMENT((#38025));
#38025=SURFACE_STYLE_USAGE(.BOTH.,#38027);
#38027=SURFACE_SIDE_STYLE('',(#38029));
#38029=SURFACE_STYLE_FILL_AREA(#38031);
#38031=FILL_AREA_STYLE('Opaque(202,209,238)',(#38033));
#38033=FILL_AREA_STYLE_COLOUR('Opaque(202,209,238)',#38035);
#38035=COLOUR_RGB('Opaque(202,209,238)', 0.66274510, 0.83137255, 0.94901961);
ENDSEC;
END-ISO-10303-21;
